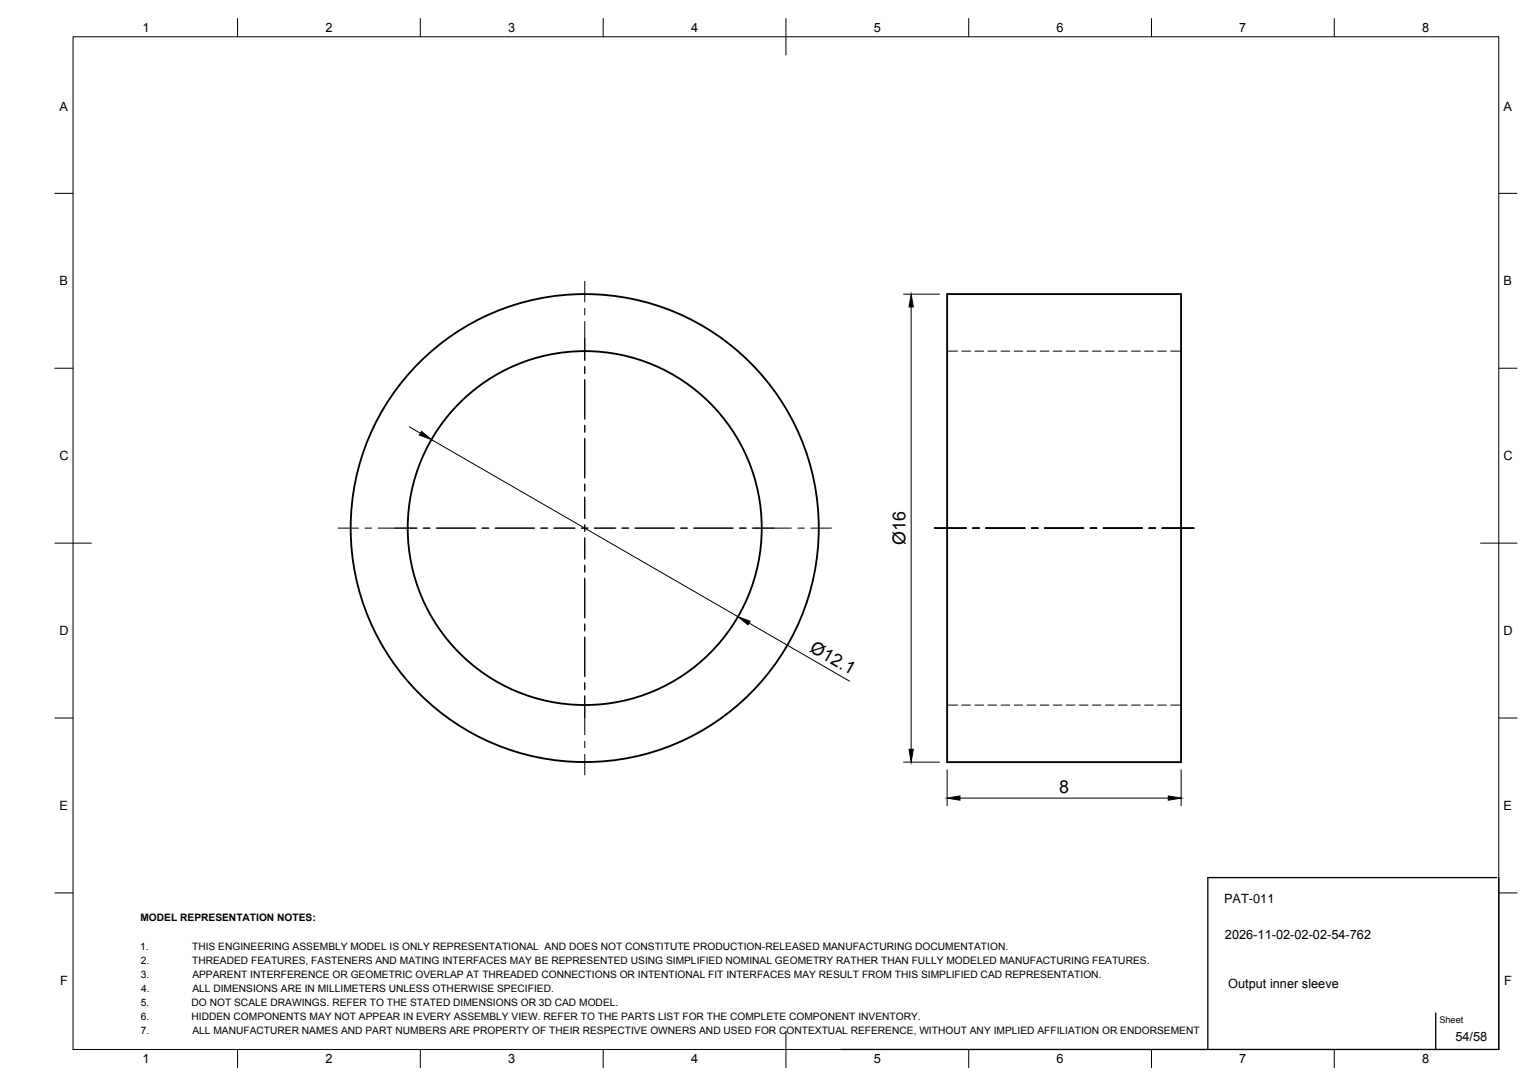
ISO-10303-21;
HEADER;
/* Generated by software containing ST-Developer
 * from STEP Tools, Inc. (www.steptools.com) 
 */

FILE_DESCRIPTION(
/* description */ ('Belt tension measurement rig'),
/* implementation_level */ '2;1');

FILE_NAME(
/* name */ 'Output inner sleeve.step',
/* time_stamp */ '2026-10-28T03:24:44-07:00',
/* author */ (''),
/* organization */ (''),
/* preprocessor_version */ 'ST-DEVELOPER v20.2',
/* originating_system */ 'Autodesk Translation Framework v15.17.0.0',
/* authorisation */ '');

FILE_SCHEMA (('AUTOMOTIVE_DESIGN { 1 0 10303 214 3 1 1 }'));
ENDSEC;

DATA;
#10=MECHANICAL_DESIGN_GEOMETRIC_PRESENTATION_REPRESENTATION('',(#753),#23587);
#628=SHAPE_REPRESENTATION_RELATIONSHIP('SRR','None',#23879,#683);
#683=ADVANCED_BREP_SHAPE_REPRESENTATION('',(#821),#23577);
#753=STYLED_ITEM('',(#24204),#821);
#821=MANIFOLD_SOLID_BREP('Body1',#12260);
#1011=FACE_BOUND('',#2785,.T.);
#1012=FACE_BOUND('',#2787,.T.);
#1306=PLANE('',#14048);
#1307=PLANE('',#14049);
#1896=FACE_OUTER_BOUND('',#2782,.T.);
#1897=FACE_OUTER_BOUND('',#2783,.T.);
#1898=FACE_OUTER_BOUND('',#2784,.T.);
#1899=FACE_OUTER_BOUND('',#2786,.T.);
#2782=EDGE_LOOP('',(#10360,#10361,#10362,#10363));
#2783=EDGE_LOOP('',(#10364,#10365,#10366,#10367));
#2784=EDGE_LOOP('',(#10368));
#2785=EDGE_LOOP('',(#10369));
#2786=EDGE_LOOP('',(#10370));
#2787=EDGE_LOOP('',(#10371));
#3563=LINE('',#22202,#4314);
#3564=LINE('',#22208,#4315);
#4314=VECTOR('',#17448,0.605);
#4315=VECTOR('',#17455,0.800000000000001);
#5024=CIRCLE('',#14043,0.605);
#5025=CIRCLE('',#14044,0.605);
#5026=CIRCLE('',#14046,0.800000000000001);
#5027=CIRCLE('',#14047,0.800000000000001);
#6061=VERTEX_POINT('',#22199);
#6062=VERTEX_POINT('',#22201);
#6063=VERTEX_POINT('',#22205);
#6064=VERTEX_POINT('',#22207);
#7539=EDGE_CURVE('',#6061,#6061,#5024,.T.);
#7540=EDGE_CURVE('',#6061,#6062,#3563,.T.);
#7541=EDGE_CURVE('',#6062,#6062,#5025,.T.);
#7542=EDGE_CURVE('',#6063,#6063,#5026,.T.);
#7543=EDGE_CURVE('',#6063,#6064,#3564,.T.);
#7544=EDGE_CURVE('',#6064,#6064,#5027,.T.);
#10360=ORIENTED_EDGE('',*,*,#7539,.F.);
#10361=ORIENTED_EDGE('',*,*,#7540,.T.);
#10362=ORIENTED_EDGE('',*,*,#7541,.T.);
#10363=ORIENTED_EDGE('',*,*,#7540,.F.);
#10364=ORIENTED_EDGE('',*,*,#7542,.F.);
#10365=ORIENTED_EDGE('',*,*,#7543,.T.);
#10366=ORIENTED_EDGE('',*,*,#7544,.T.);
#10367=ORIENTED_EDGE('',*,*,#7543,.F.);
#10368=ORIENTED_EDGE('',*,*,#7542,.T.);
#10369=ORIENTED_EDGE('',*,*,#7539,.T.);
#10370=ORIENTED_EDGE('',*,*,#7544,.F.);
#10371=ORIENTED_EDGE('',*,*,#7541,.F.);
#11385=CYLINDRICAL_SURFACE('',#14042,0.605);
#11386=CYLINDRICAL_SURFACE('',#14045,0.800000000000001);
#12037=ADVANCED_FACE('',(#1896),#11385,.F.);
#12038=ADVANCED_FACE('',(#1897),#11386,.T.);
#12039=ADVANCED_FACE('',(#1898,#1011),#1306,.T.);
#12040=ADVANCED_FACE('',(#1899,#1012),#1307,.F.);
#12260=CLOSED_SHELL('',(#12037,#12038,#12039,#12040));
#14041=AXIS2_PLACEMENT_3D('',#22197,#17442,#17443);
#14042=AXIS2_PLACEMENT_3D('',#22198,#17444,#17445);
#14043=AXIS2_PLACEMENT_3D('',#22200,#17446,#17447);
#14044=AXIS2_PLACEMENT_3D('',#22203,#17449,#17450);
#14045=AXIS2_PLACEMENT_3D('',#22204,#17451,#17452);
#14046=AXIS2_PLACEMENT_3D('',#22206,#17453,#17454);
#14047=AXIS2_PLACEMENT_3D('',#22209,#17456,#17457);
#14048=AXIS2_PLACEMENT_3D('',#22210,#17458,#17459);
#14049=AXIS2_PLACEMENT_3D('',#22211,#17460,#17461);
#17442=DIRECTION('axis',(0.,0.,1.));
#17443=DIRECTION('refdir',(1.,0.,0.));
#17444=DIRECTION('center_axis',(0.,1.,0.));
#17445=DIRECTION('ref_axis',(1.,0.,0.));
#17446=DIRECTION('center_axis',(0.,-1.,0.));
#17447=DIRECTION('ref_axis',(1.,0.,0.));
#17448=DIRECTION('',(0.,-1.,0.));
#17449=DIRECTION('center_axis',(0.,-1.,0.));
#17450=DIRECTION('ref_axis',(1.,0.,0.));
#17451=DIRECTION('center_axis',(0.,1.,0.));
#17452=DIRECTION('ref_axis',(1.,0.,0.));
#17453=DIRECTION('center_axis',(0.,1.,0.));
#17454=DIRECTION('ref_axis',(1.,0.,0.));
#17455=DIRECTION('',(0.,-1.,0.));
#17456=DIRECTION('center_axis',(0.,1.,0.));
#17457=DIRECTION('ref_axis',(1.,0.,0.));
#17458=DIRECTION('center_axis',(0.,1.,0.));
#17459=DIRECTION('ref_axis',(1.,0.,0.));
#17460=DIRECTION('center_axis',(0.,1.,0.));
#17461=DIRECTION('ref_axis',(1.,0.,0.));
#22197=CARTESIAN_POINT('',(0.,0.,0.));
#22198=CARTESIAN_POINT('Origin',(10.,-0.4,7.));
#22199=CARTESIAN_POINT('',(9.395,0.4,7.));
#22200=CARTESIAN_POINT('Origin',(10.,0.4,7.));
#22201=CARTESIAN_POINT('',(9.395,-0.4,7.));
#22202=CARTESIAN_POINT('',(9.395,-0.4,7.));
#22203=CARTESIAN_POINT('Origin',(10.,-0.4,7.));
#22204=CARTESIAN_POINT('Origin',(10.,-0.4,7.));
#22205=CARTESIAN_POINT('',(9.2,0.4,7.));
#22206=CARTESIAN_POINT('Origin',(10.,0.4,7.));
#22207=CARTESIAN_POINT('',(9.2,-0.4,7.));
#22208=CARTESIAN_POINT('',(9.2,-0.4,7.));
#22209=CARTESIAN_POINT('Origin',(10.,-0.4,7.));
#22210=CARTESIAN_POINT('Origin',(10.,0.4,7.));
#22211=CARTESIAN_POINT('Origin',(10.,-0.4,7.));
#23512=UNCERTAINTY_MEASURE_WITH_UNIT(LENGTH_MEASURE(0.001),#23588,
'DISTANCE_ACCURACY_VALUE',
'Maximum model space distance between geometric entities at asserted c
onnectivities');
#23522=UNCERTAINTY_MEASURE_WITH_UNIT(LENGTH_MEASURE(0.001),#23588,
'DISTANCE_ACCURACY_VALUE',
'Maximum model space distance between geometric entities at asserted c
onnectivities');
#23577=(
GEOMETRIC_REPRESENTATION_CONTEXT(3)
GLOBAL_UNCERTAINTY_ASSIGNED_CONTEXT((#23512))
GLOBAL_UNIT_ASSIGNED_CONTEXT((#23588,#23590,#23591))
REPRESENTATION_CONTEXT('','3D')
);
#23587=(
GEOMETRIC_REPRESENTATION_CONTEXT(3)
GLOBAL_UNCERTAINTY_ASSIGNED_CONTEXT((#23522))
GLOBAL_UNIT_ASSIGNED_CONTEXT((#23588,#23590,#23591))
REPRESENTATION_CONTEXT('','3D')
);
#23588=(
LENGTH_UNIT()
NAMED_UNIT(*)
SI_UNIT(.CENTI.,.METRE.)
);
#23590=(
NAMED_UNIT(*)
PLANE_ANGLE_UNIT()
SI_UNIT($,.RADIAN.)
);
#23591=(
NAMED_UNIT(*)
SI_UNIT($,.STERADIAN.)
SOLID_ANGLE_UNIT()
);
#23646=SHAPE_DEFINITION_REPRESENTATION(#23723,#23879);
#23723=PRODUCT_DEFINITION_SHAPE('',$,#23944);
#23879=SHAPE_REPRESENTATION('',(#14041),#23577);
#23889=PRODUCT_DEFINITION_CONTEXT('part definition',#24083,'design');
#23944=PRODUCT_DEFINITION('Output inner sleeve','Output inner sleeve',#24008,
#23889);
#24008=PRODUCT_DEFINITION_FORMATION('',$,#24139);
#24083=APPLICATION_CONTEXT(
'Core Data for Automotive Mechanical Design Process');
#24084=PRODUCT_CONTEXT('part definition',#24083,'mechanical');
#24139=PRODUCT('Output inner sleeve','Output inner sleeve',
'Output inner sleeve',(#24084));
#24198=COLOUR_RGB('Sky Blue',0.24,0.69,0.87);
#24199=FILL_AREA_STYLE_COLOUR('',#24198);
#24200=FILL_AREA_STYLE('',(#24199));
#24201=SURFACE_STYLE_FILL_AREA(#24200);
#24202=SURFACE_SIDE_STYLE('',(#24201));
#24203=SURFACE_STYLE_USAGE(.BOTH.,#24202);
#24204=PRESENTATION_STYLE_ASSIGNMENT((#24203));
ENDSEC;
END-ISO-10303-21;
